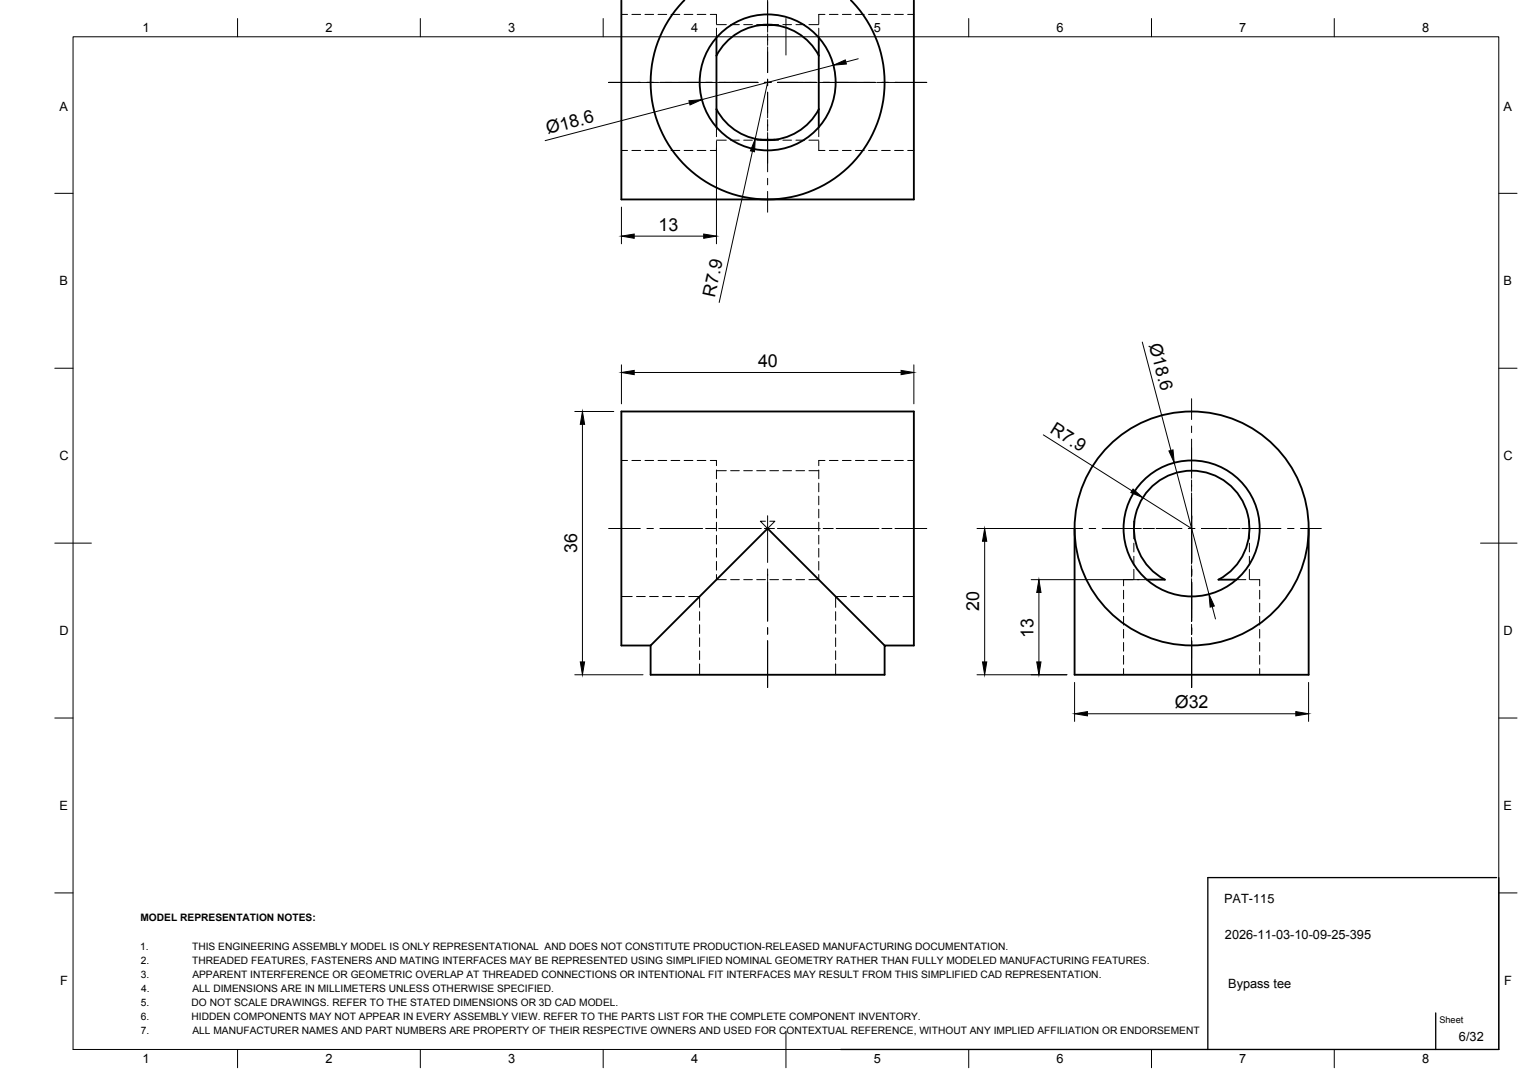
ISO-10303-21;
HEADER;
/* Generated by software containing ST-Developer
 * from STEP Tools, Inc. (www.steptools.com) 
 */

FILE_DESCRIPTION(
/* description */ ('Union bypass pipe loop'),
/* implementation_level */ '2;1');

FILE_NAME(
/* name */ 'Bypass tee.step',
/* time_stamp */ '2026-10-27T21:00:29-07:00',
/* author */ (''),
/* organization */ (''),
/* preprocessor_version */ 'ST-DEVELOPER v20.2',
/* originating_system */ 'Autodesk Translation Framework v15.17.0.0',
/* authorisation */ '');

FILE_SCHEMA (('AUTOMOTIVE_DESIGN { 1 0 10303 214 3 1 1 }'));
ENDSEC;

DATA;
#10=MECHANICAL_DESIGN_GEOMETRIC_PRESENTATION_REPRESENTATION('',(#460),#10095);
#11=ELLIPSE('',#6238,1.31521861300698,0.93);
#12=ELLIPSE('',#6239,1.31521861300698,0.93);
#13=ELLIPSE('',#6241,1.31521861300698,0.93);
#14=ELLIPSE('',#6249,1.11722871427474,0.789999999999999);
#15=ELLIPSE('',#6250,1.11722871427474,0.789999999999999);
#16=ELLIPSE('',#6254,1.11722871427474,0.789999999999999);
#17=ELLIPSE('',#6255,1.11722871427474,0.789999999999999);
#18=ELLIPSE('',#6263,1.11722871427474,0.789999999999999);
#19=ELLIPSE('',#6264,1.11722871427474,0.789999999999999);
#20=ELLIPSE('',#6265,1.11722871427474,0.789999999999999);
#21=ELLIPSE('',#6266,1.11722871427474,0.789999999999999);
#22=ELLIPSE('',#6274,2.26274169979695,1.6);
#23=ELLIPSE('',#6275,2.26274169979695,1.6);
#24=ELLIPSE('',#6277,2.26274169979695,1.6);
#396=SHAPE_REPRESENTATION_RELATIONSHIP('SRR','None',#10265,#428);
#428=ADVANCED_BREP_SHAPE_REPRESENTATION('',(#490),#10077);
#460=STYLED_ITEM('',(#10493),#490);
#490=MANIFOLD_SOLID_BREP('Body1',#5533);
#579=FACE_BOUND('',#1404,.T.);
#580=FACE_BOUND('',#1407,.T.);
#581=FACE_BOUND('',#1409,.T.);
#723=PLANE('',#6233);
#724=PLANE('',#6242);
#725=PLANE('',#6251);
#726=PLANE('',#6256);
#727=PLANE('',#6267);
#728=PLANE('',#6272);
#729=PLANE('',#6278);
#730=PLANE('',#6282);
#731=PLANE('',#6283);
#988=FACE_OUTER_BOUND('',#1388,.T.);
#989=FACE_OUTER_BOUND('',#1389,.T.);
#990=FACE_OUTER_BOUND('',#1390,.T.);
#991=FACE_OUTER_BOUND('',#1391,.T.);
#992=FACE_OUTER_BOUND('',#1392,.T.);
#993=FACE_OUTER_BOUND('',#1393,.T.);
#994=FACE_OUTER_BOUND('',#1394,.T.);
#995=FACE_OUTER_BOUND('',#1395,.T.);
#996=FACE_OUTER_BOUND('',#1396,.T.);
#997=FACE_OUTER_BOUND('',#1397,.T.);
#998=FACE_OUTER_BOUND('',#1398,.T.);
#999=FACE_OUTER_BOUND('',#1399,.T.);
#1000=FACE_OUTER_BOUND('',#1400,.T.);
#1001=FACE_OUTER_BOUND('',#1401,.T.);
#1002=FACE_OUTER_BOUND('',#1402,.T.);
#1003=FACE_OUTER_BOUND('',#1403,.T.);
#1004=FACE_OUTER_BOUND('',#1405,.T.);
#1005=FACE_OUTER_BOUND('',#1406,.T.);
#1006=FACE_OUTER_BOUND('',#1408,.T.);
#1388=EDGE_LOOP('',(#4352,#4353,#4354,#4355));
#1389=EDGE_LOOP('',(#4356,#4357,#4358,#4359,#4360,#4361,#4362,#4363));
#1390=EDGE_LOOP('',(#4364,#4365,#4366,#4367));
#1391=EDGE_LOOP('',(#4368,#4369,#4370,#4371,#4372,#4373));
#1392=EDGE_LOOP('',(#4374,#4375,#4376));
#1393=EDGE_LOOP('',(#4377,#4378,#4379,#4380,#4381));
#1394=EDGE_LOOP('',(#4382,#4383,#4384));
#1395=EDGE_LOOP('',(#4385,#4386,#4387,#4388,#4389));
#1396=EDGE_LOOP('',(#4390,#4391,#4392,#4393,#4394,#4395,#4396));
#1397=EDGE_LOOP('',(#4397,#4398,#4399,#4400,#4401,#4402,#4403,#4404,#4405,
#4406,#4407,#4408));
#1398=EDGE_LOOP('',(#4409,#4410));
#1399=EDGE_LOOP('',(#4411,#4412,#4413));
#1400=EDGE_LOOP('',(#4414,#4415,#4416));
#1401=EDGE_LOOP('',(#4417,#4418));
#1402=EDGE_LOOP('',(#4419,#4420,#4421,#4422,#4423,#4424));
#1403=EDGE_LOOP('',(#4425));
#1404=EDGE_LOOP('',(#4426));
#1405=EDGE_LOOP('',(#4427,#4428,#4429,#4430,#4431,#4432,#4433,#4434,#4435));
#1406=EDGE_LOOP('',(#4436));
#1407=EDGE_LOOP('',(#4437));
#1408=EDGE_LOOP('',(#4438));
#1409=EDGE_LOOP('',(#4439));
#1797=LINE('',#9166,#2173);
#1798=LINE('',#9170,#2174);
#1799=LINE('',#9176,#2175);
#1800=LINE('',#9185,#2176);
#1801=LINE('',#9188,#2177);
#1802=LINE('',#9193,#2178);
#1803=LINE('',#9214,#2179);
#1804=LINE('',#9219,#2180);
#1805=LINE('',#9224,#2181);
#1806=LINE('',#9239,#2182);
#1807=LINE('',#9246,#2183);
#1808=LINE('',#9248,#2184);
#2173=VECTOR('',#7451,1.);
#2174=VECTOR('',#7454,1.);
#2175=VECTOR('',#7461,0.93);
#2176=VECTOR('',#7472,1.);
#2177=VECTOR('',#7475,1.);
#2178=VECTOR('',#7480,0.93);
#2179=VECTOR('',#7513,0.93);
#2180=VECTOR('',#7518,1.);
#2181=VECTOR('',#7523,1.);
#2182=VECTOR('',#7544,1.6);
#2183=VECTOR('',#7555,1.6);
#2184=VECTOR('',#7556,1.6);
#2496=CIRCLE('',#6234,0.93);
#2497=CIRCLE('',#6235,0.789999999999999);
#2498=CIRCLE('',#6237,0.93);
#2499=CIRCLE('',#6240,0.93);
#2500=CIRCLE('',#6243,0.789999999999999);
#2501=CIRCLE('',#6245,0.93);
#2502=CIRCLE('',#6246,0.93);
#2503=CIRCLE('',#6247,0.93);
#2504=CIRCLE('',#6252,0.79);
#2505=CIRCLE('',#6257,0.79);
#2506=CIRCLE('',#6258,0.93);
#2507=CIRCLE('',#6259,0.93);
#2508=CIRCLE('',#6261,0.93);
#2509=CIRCLE('',#6268,0.789999999999999);
#2510=CIRCLE('',#6270,0.789999999999999);
#2511=CIRCLE('',#6276,1.6);
#2512=CIRCLE('',#6280,1.6);
#2513=CIRCLE('',#6281,1.6);
#2832=VERTEX_POINT('',#9164);
#2833=VERTEX_POINT('',#9165);
#2834=VERTEX_POINT('',#9167);
#2835=VERTEX_POINT('',#9169);
#2836=VERTEX_POINT('',#9173);
#2837=VERTEX_POINT('',#9175);
#2838=VERTEX_POINT('',#9178);
#2839=VERTEX_POINT('',#9180);
#2840=VERTEX_POINT('',#9184);
#2841=VERTEX_POINT('',#9186);
#2842=VERTEX_POINT('',#9190);
#2843=VERTEX_POINT('',#9192);
#2844=VERTEX_POINT('',#9197);
#2845=VERTEX_POINT('',#9203);
#2846=VERTEX_POINT('',#9208);
#2847=VERTEX_POINT('',#9212);
#2848=VERTEX_POINT('',#9216);
#2849=VERTEX_POINT('',#9218);
#2850=VERTEX_POINT('',#9221);
#2851=VERTEX_POINT('',#9223);
#2852=VERTEX_POINT('',#9233);
#2853=VERTEX_POINT('',#9234);
#2854=VERTEX_POINT('',#9236);
#2855=VERTEX_POINT('',#9238);
#2856=VERTEX_POINT('',#9244);
#2857=VERTEX_POINT('',#9247);
#3374=EDGE_CURVE('',#2832,#2833,#1797,.T.);
#3375=EDGE_CURVE('',#2834,#2832,#2496,.T.);
#3376=EDGE_CURVE('',#2835,#2834,#1798,.T.);
#3377=EDGE_CURVE('',#2833,#2835,#2497,.T.);
#3378=EDGE_CURVE('',#2836,#2836,#2498,.T.);
#3379=EDGE_CURVE('',#2836,#2837,#1799,.T.);
#3380=EDGE_CURVE('',#2834,#2837,#11,.T.);
#3381=EDGE_CURVE('',#2838,#2832,#12,.T.);
#3382=EDGE_CURVE('',#2838,#2839,#2499,.T.);
#3383=EDGE_CURVE('',#2837,#2839,#13,.T.);
#3384=EDGE_CURVE('',#2840,#2838,#1800,.T.);
#3385=EDGE_CURVE('',#2841,#2840,#2500,.T.);
#3386=EDGE_CURVE('',#2839,#2841,#1801,.T.);
#3387=EDGE_CURVE('',#2842,#2832,#2501,.T.);
#3388=EDGE_CURVE('',#2842,#2843,#1802,.T.);
#3389=EDGE_CURVE('',#2843,#2843,#2502,.T.);
#3390=EDGE_CURVE('',#2838,#2842,#2503,.T.);
#3391=EDGE_CURVE('',#2844,#2835,#14,.T.);
#3392=EDGE_CURVE('',#2833,#2844,#15,.T.);
#3393=EDGE_CURVE('',#2840,#2833,#2504,.T.);
#3394=EDGE_CURVE('',#2845,#2840,#16,.T.);
#3395=EDGE_CURVE('',#2841,#2845,#17,.T.);
#3396=EDGE_CURVE('',#2835,#2841,#2505,.T.);
#3397=EDGE_CURVE('',#2846,#2834,#2506,.T.);
#3398=EDGE_CURVE('',#2839,#2846,#2507,.T.);
#3399=EDGE_CURVE('',#2847,#2847,#2508,.T.);
#3400=EDGE_CURVE('',#2847,#2846,#1803,.T.);
#3401=EDGE_CURVE('',#2844,#2848,#18,.T.);
#3402=EDGE_CURVE('',#2848,#2849,#1804,.T.);
#3403=EDGE_CURVE('',#2849,#2844,#19,.T.);
#3404=EDGE_CURVE('',#2845,#2850,#20,.T.);
#3405=EDGE_CURVE('',#2850,#2851,#1805,.T.);
#3406=EDGE_CURVE('',#2851,#2845,#21,.T.);
#3407=EDGE_CURVE('',#2851,#2850,#2509,.T.);
#3408=EDGE_CURVE('',#2849,#2848,#2510,.T.);
#3409=EDGE_CURVE('',#2852,#2853,#22,.T.);
#3410=EDGE_CURVE('',#2854,#2852,#23,.T.);
#3411=EDGE_CURVE('',#2854,#2855,#1806,.T.);
#3412=EDGE_CURVE('',#2855,#2855,#2511,.T.);
#3413=EDGE_CURVE('',#2853,#2854,#24,.T.);
#3414=EDGE_CURVE('',#2856,#2856,#2512,.T.);
#3415=EDGE_CURVE('',#2856,#2852,#1807,.T.);
#3416=EDGE_CURVE('',#2852,#2857,#1808,.T.);
#3417=EDGE_CURVE('',#2857,#2857,#2513,.T.);
#4352=ORIENTED_EDGE('',*,*,#3374,.F.);
#4353=ORIENTED_EDGE('',*,*,#3375,.F.);
#4354=ORIENTED_EDGE('',*,*,#3376,.F.);
#4355=ORIENTED_EDGE('',*,*,#3377,.F.);
#4356=ORIENTED_EDGE('',*,*,#3378,.F.);
#4357=ORIENTED_EDGE('',*,*,#3379,.T.);
#4358=ORIENTED_EDGE('',*,*,#3380,.F.);
#4359=ORIENTED_EDGE('',*,*,#3375,.T.);
#4360=ORIENTED_EDGE('',*,*,#3381,.F.);
#4361=ORIENTED_EDGE('',*,*,#3382,.T.);
#4362=ORIENTED_EDGE('',*,*,#3383,.F.);
#4363=ORIENTED_EDGE('',*,*,#3379,.F.);
#4364=ORIENTED_EDGE('',*,*,#3384,.F.);
#4365=ORIENTED_EDGE('',*,*,#3385,.F.);
#4366=ORIENTED_EDGE('',*,*,#3386,.F.);
#4367=ORIENTED_EDGE('',*,*,#3382,.F.);
#4368=ORIENTED_EDGE('',*,*,#3381,.T.);
#4369=ORIENTED_EDGE('',*,*,#3387,.F.);
#4370=ORIENTED_EDGE('',*,*,#3388,.T.);
#4371=ORIENTED_EDGE('',*,*,#3389,.F.);
#4372=ORIENTED_EDGE('',*,*,#3388,.F.);
#4373=ORIENTED_EDGE('',*,*,#3390,.F.);
#4374=ORIENTED_EDGE('',*,*,#3377,.T.);
#4375=ORIENTED_EDGE('',*,*,#3391,.F.);
#4376=ORIENTED_EDGE('',*,*,#3392,.F.);
#4377=ORIENTED_EDGE('',*,*,#3384,.T.);
#4378=ORIENTED_EDGE('',*,*,#3390,.T.);
#4379=ORIENTED_EDGE('',*,*,#3387,.T.);
#4380=ORIENTED_EDGE('',*,*,#3374,.T.);
#4381=ORIENTED_EDGE('',*,*,#3393,.F.);
#4382=ORIENTED_EDGE('',*,*,#3385,.T.);
#4383=ORIENTED_EDGE('',*,*,#3394,.F.);
#4384=ORIENTED_EDGE('',*,*,#3395,.F.);
#4385=ORIENTED_EDGE('',*,*,#3386,.T.);
#4386=ORIENTED_EDGE('',*,*,#3396,.F.);
#4387=ORIENTED_EDGE('',*,*,#3376,.T.);
#4388=ORIENTED_EDGE('',*,*,#3397,.F.);
#4389=ORIENTED_EDGE('',*,*,#3398,.F.);
#4390=ORIENTED_EDGE('',*,*,#3399,.F.);
#4391=ORIENTED_EDGE('',*,*,#3400,.T.);
#4392=ORIENTED_EDGE('',*,*,#3397,.T.);
#4393=ORIENTED_EDGE('',*,*,#3380,.T.);
#4394=ORIENTED_EDGE('',*,*,#3383,.T.);
#4395=ORIENTED_EDGE('',*,*,#3398,.T.);
#4396=ORIENTED_EDGE('',*,*,#3400,.F.);
#4397=ORIENTED_EDGE('',*,*,#3393,.T.);
#4398=ORIENTED_EDGE('',*,*,#3392,.T.);
#4399=ORIENTED_EDGE('',*,*,#3401,.T.);
#4400=ORIENTED_EDGE('',*,*,#3402,.T.);
#4401=ORIENTED_EDGE('',*,*,#3403,.T.);
#4402=ORIENTED_EDGE('',*,*,#3391,.T.);
#4403=ORIENTED_EDGE('',*,*,#3396,.T.);
#4404=ORIENTED_EDGE('',*,*,#3395,.T.);
#4405=ORIENTED_EDGE('',*,*,#3404,.T.);
#4406=ORIENTED_EDGE('',*,*,#3405,.T.);
#4407=ORIENTED_EDGE('',*,*,#3406,.T.);
#4408=ORIENTED_EDGE('',*,*,#3394,.T.);
#4409=ORIENTED_EDGE('',*,*,#3405,.F.);
#4410=ORIENTED_EDGE('',*,*,#3407,.F.);
#4411=ORIENTED_EDGE('',*,*,#3403,.F.);
#4412=ORIENTED_EDGE('',*,*,#3408,.T.);
#4413=ORIENTED_EDGE('',*,*,#3401,.F.);
#4414=ORIENTED_EDGE('',*,*,#3406,.F.);
#4415=ORIENTED_EDGE('',*,*,#3407,.T.);
#4416=ORIENTED_EDGE('',*,*,#3404,.F.);
#4417=ORIENTED_EDGE('',*,*,#3402,.F.);
#4418=ORIENTED_EDGE('',*,*,#3408,.F.);
#4419=ORIENTED_EDGE('',*,*,#3409,.F.);
#4420=ORIENTED_EDGE('',*,*,#3410,.F.);
#4421=ORIENTED_EDGE('',*,*,#3411,.T.);
#4422=ORIENTED_EDGE('',*,*,#3412,.T.);
#4423=ORIENTED_EDGE('',*,*,#3411,.F.);
#4424=ORIENTED_EDGE('',*,*,#3413,.F.);
#4425=ORIENTED_EDGE('',*,*,#3412,.F.);
#4426=ORIENTED_EDGE('',*,*,#3378,.T.);
#4427=ORIENTED_EDGE('',*,*,#3414,.F.);
#4428=ORIENTED_EDGE('',*,*,#3415,.T.);
#4429=ORIENTED_EDGE('',*,*,#3409,.T.);
#4430=ORIENTED_EDGE('',*,*,#3413,.T.);
#4431=ORIENTED_EDGE('',*,*,#3410,.T.);
#4432=ORIENTED_EDGE('',*,*,#3416,.T.);
#4433=ORIENTED_EDGE('',*,*,#3417,.T.);
#4434=ORIENTED_EDGE('',*,*,#3416,.F.);
#4435=ORIENTED_EDGE('',*,*,#3415,.F.);
#4436=ORIENTED_EDGE('',*,*,#3414,.T.);
#4437=ORIENTED_EDGE('',*,*,#3389,.T.);
#4438=ORIENTED_EDGE('',*,*,#3417,.F.);
#4439=ORIENTED_EDGE('',*,*,#3399,.T.);
#5131=CYLINDRICAL_SURFACE('',#6236,0.93);
#5132=CYLINDRICAL_SURFACE('',#6244,0.93);
#5133=CYLINDRICAL_SURFACE('',#6248,0.789999999999999);
#5134=CYLINDRICAL_SURFACE('',#6253,0.789999999999999);
#5135=CYLINDRICAL_SURFACE('',#6260,0.93);
#5136=CYLINDRICAL_SURFACE('',#6262,0.79);
#5137=CYLINDRICAL_SURFACE('',#6269,0.789999999999999);
#5138=CYLINDRICAL_SURFACE('',#6271,0.789999999999999);
#5139=CYLINDRICAL_SURFACE('',#6273,1.6);
#5140=CYLINDRICAL_SURFACE('',#6279,1.6);
#5337=ADVANCED_FACE('',(#988),#723,.F.);
#5338=ADVANCED_FACE('',(#989),#5131,.F.);
#5339=ADVANCED_FACE('',(#990),#724,.F.);
#5340=ADVANCED_FACE('',(#991),#5132,.F.);
#5341=ADVANCED_FACE('',(#992),#5133,.F.);
#5342=ADVANCED_FACE('',(#993),#725,.T.);
#5343=ADVANCED_FACE('',(#994),#5134,.F.);
#5344=ADVANCED_FACE('',(#995),#726,.F.);
#5345=ADVANCED_FACE('',(#996),#5135,.F.);
#5346=ADVANCED_FACE('',(#997),#5136,.F.);
#5347=ADVANCED_FACE('',(#998),#727,.F.);
#5348=ADVANCED_FACE('',(#999),#5137,.F.);
#5349=ADVANCED_FACE('',(#1000),#5138,.F.);
#5350=ADVANCED_FACE('',(#1001),#728,.F.);
#5351=ADVANCED_FACE('',(#1002),#5139,.T.);
#5352=ADVANCED_FACE('',(#1003,#579),#729,.F.);
#5353=ADVANCED_FACE('',(#1004),#5140,.T.);
#5354=ADVANCED_FACE('',(#1005,#580),#730,.T.);
#5355=ADVANCED_FACE('',(#1006,#581),#731,.F.);
#5533=CLOSED_SHELL('',(#5337,#5338,#5339,#5340,#5341,#5342,#5343,#5344,
#5345,#5346,#5347,#5348,#5349,#5350,#5351,#5352,#5353,#5354,#5355));
#6232=AXIS2_PLACEMENT_3D('',#9162,#7447,#7448);
#6233=AXIS2_PLACEMENT_3D('',#9163,#7449,#7450);
#6234=AXIS2_PLACEMENT_3D('',#9168,#7452,#7453);
#6235=AXIS2_PLACEMENT_3D('',#9171,#7455,#7456);
#6236=AXIS2_PLACEMENT_3D('',#9172,#7457,#7458);
#6237=AXIS2_PLACEMENT_3D('',#9174,#7459,#7460);
#6238=AXIS2_PLACEMENT_3D('',#9177,#7462,#7463);
#6239=AXIS2_PLACEMENT_3D('',#9179,#7464,#7465);
#6240=AXIS2_PLACEMENT_3D('',#9181,#7466,#7467);
#6241=AXIS2_PLACEMENT_3D('',#9182,#7468,#7469);
#6242=AXIS2_PLACEMENT_3D('',#9183,#7470,#7471);
#6243=AXIS2_PLACEMENT_3D('',#9187,#7473,#7474);
#6244=AXIS2_PLACEMENT_3D('',#9189,#7476,#7477);
#6245=AXIS2_PLACEMENT_3D('',#9191,#7478,#7479);
#6246=AXIS2_PLACEMENT_3D('',#9194,#7481,#7482);
#6247=AXIS2_PLACEMENT_3D('',#9195,#7483,#7484);
#6248=AXIS2_PLACEMENT_3D('',#9196,#7485,#7486);
#6249=AXIS2_PLACEMENT_3D('',#9198,#7487,#7488);
#6250=AXIS2_PLACEMENT_3D('',#9199,#7489,#7490);
#6251=AXIS2_PLACEMENT_3D('',#9200,#7491,#7492);
#6252=AXIS2_PLACEMENT_3D('',#9201,#7493,#7494);
#6253=AXIS2_PLACEMENT_3D('',#9202,#7495,#7496);
#6254=AXIS2_PLACEMENT_3D('',#9204,#7497,#7498);
#6255=AXIS2_PLACEMENT_3D('',#9205,#7499,#7500);
#6256=AXIS2_PLACEMENT_3D('',#9206,#7501,#7502);
#6257=AXIS2_PLACEMENT_3D('',#9207,#7503,#7504);
#6258=AXIS2_PLACEMENT_3D('',#9209,#7505,#7506);
#6259=AXIS2_PLACEMENT_3D('',#9210,#7507,#7508);
#6260=AXIS2_PLACEMENT_3D('',#9211,#7509,#7510);
#6261=AXIS2_PLACEMENT_3D('',#9213,#7511,#7512);
#6262=AXIS2_PLACEMENT_3D('',#9215,#7514,#7515);
#6263=AXIS2_PLACEMENT_3D('',#9217,#7516,#7517);
#6264=AXIS2_PLACEMENT_3D('',#9220,#7519,#7520);
#6265=AXIS2_PLACEMENT_3D('',#9222,#7521,#7522);
#6266=AXIS2_PLACEMENT_3D('',#9225,#7524,#7525);
#6267=AXIS2_PLACEMENT_3D('',#9226,#7526,#7527);
#6268=AXIS2_PLACEMENT_3D('',#9227,#7528,#7529);
#6269=AXIS2_PLACEMENT_3D('',#9228,#7530,#7531);
#6270=AXIS2_PLACEMENT_3D('',#9229,#7532,#7533);
#6271=AXIS2_PLACEMENT_3D('',#9230,#7534,#7535);
#6272=AXIS2_PLACEMENT_3D('',#9231,#7536,#7537);
#6273=AXIS2_PLACEMENT_3D('',#9232,#7538,#7539);
#6274=AXIS2_PLACEMENT_3D('',#9235,#7540,#7541);
#6275=AXIS2_PLACEMENT_3D('',#9237,#7542,#7543);
#6276=AXIS2_PLACEMENT_3D('',#9240,#7545,#7546);
#6277=AXIS2_PLACEMENT_3D('',#9241,#7547,#7548);
#6278=AXIS2_PLACEMENT_3D('',#9242,#7549,#7550);
#6279=AXIS2_PLACEMENT_3D('',#9243,#7551,#7552);
#6280=AXIS2_PLACEMENT_3D('',#9245,#7553,#7554);
#6281=AXIS2_PLACEMENT_3D('',#9249,#7557,#7558);
#6282=AXIS2_PLACEMENT_3D('',#9250,#7559,#7560);
#6283=AXIS2_PLACEMENT_3D('',#9251,#7561,#7562);
#7447=DIRECTION('axis',(0.,0.,1.));
#7448=DIRECTION('refdir',(1.,0.,0.));
#7449=DIRECTION('center_axis',(0.,1.,0.));
#7450=DIRECTION('ref_axis',(1.,0.,0.));
#7451=DIRECTION('',(0.,0.,-1.));
#7452=DIRECTION('center_axis',(0.,1.,0.));
#7453=DIRECTION('ref_axis',(1.,0.,0.));
#7454=DIRECTION('',(0.,0.,1.));
#7455=DIRECTION('center_axis',(0.,-1.,0.));
#7456=DIRECTION('ref_axis',(1.,0.,0.));
#7457=DIRECTION('center_axis',(0.,1.,0.));
#7458=DIRECTION('ref_axis',(1.,0.,0.));
#7459=DIRECTION('center_axis',(0.,1.,0.));
#7460=DIRECTION('ref_axis',(1.,0.,0.));
#7461=DIRECTION('',(0.,1.,0.));
#7462=DIRECTION('center_axis',(0.707106781186548,-0.707106781186548,0.));
#7463=DIRECTION('ref_axis',(0.707106781186547,0.707106781186547,0.));
#7464=DIRECTION('center_axis',(-0.707106781186548,-0.707106781186548,0.));
#7465=DIRECTION('ref_axis',(0.707106781186547,-0.707106781186547,0.));
#7466=DIRECTION('center_axis',(0.,1.,0.));
#7467=DIRECTION('ref_axis',(1.,0.,0.));
#7468=DIRECTION('center_axis',(0.707106781186548,-0.707106781186548,0.));
#7469=DIRECTION('ref_axis',(0.707106781186547,0.707106781186547,0.));
#7470=DIRECTION('center_axis',(0.,1.,0.));
#7471=DIRECTION('ref_axis',(1.,0.,0.));
#7472=DIRECTION('',(0.,0.,-1.));
#7473=DIRECTION('center_axis',(0.,-1.,0.));
#7474=DIRECTION('ref_axis',(1.,0.,0.));
#7475=DIRECTION('',(0.,0.,1.));
#7476=DIRECTION('center_axis',(1.,0.,0.));
#7477=DIRECTION('ref_axis',(0.,0.,-1.));
#7478=DIRECTION('center_axis',(1.,0.,0.));
#7479=DIRECTION('ref_axis',(0.,0.,-1.));
#7480=DIRECTION('',(1.,0.,0.));
#7481=DIRECTION('center_axis',(-1.,0.,0.));
#7482=DIRECTION('ref_axis',(0.,0.,-1.));
#7483=DIRECTION('center_axis',(1.,0.,0.));
#7484=DIRECTION('ref_axis',(0.,0.,-1.));
#7485=DIRECTION('center_axis',(0.,1.,0.));
#7486=DIRECTION('ref_axis',(1.,0.,0.));
#7487=DIRECTION('center_axis',(0.707106781186548,-0.707106781186547,0.));
#7488=DIRECTION('ref_axis',(0.707106781186547,0.707106781186548,0.));
#7489=DIRECTION('center_axis',(-0.707106781186548,-0.707106781186547,0.));
#7490=DIRECTION('ref_axis',(0.707106781186547,-0.707106781186548,0.));
#7491=DIRECTION('center_axis',(1.,0.,0.));
#7492=DIRECTION('ref_axis',(0.,0.,-1.));
#7493=DIRECTION('center_axis',(1.,0.,0.));
#7494=DIRECTION('ref_axis',(0.,0.,-1.));
#7495=DIRECTION('center_axis',(0.,1.,0.));
#7496=DIRECTION('ref_axis',(1.,0.,0.));
#7497=DIRECTION('center_axis',(-0.707106781186548,-0.707106781186547,0.));
#7498=DIRECTION('ref_axis',(0.707106781186547,-0.707106781186548,0.));
#7499=DIRECTION('center_axis',(0.707106781186548,-0.707106781186547,0.));
#7500=DIRECTION('ref_axis',(0.707106781186547,0.707106781186548,0.));
#7501=DIRECTION('center_axis',(1.,0.,0.));
#7502=DIRECTION('ref_axis',(0.,0.,-1.));
#7503=DIRECTION('center_axis',(-1.,0.,0.));
#7504=DIRECTION('ref_axis',(0.,0.,-1.));
#7505=DIRECTION('center_axis',(1.,0.,0.));
#7506=DIRECTION('ref_axis',(0.,0.,-1.));
#7507=DIRECTION('center_axis',(1.,0.,0.));
#7508=DIRECTION('ref_axis',(0.,0.,-1.));
#7509=DIRECTION('center_axis',(1.,0.,0.));
#7510=DIRECTION('ref_axis',(0.,0.,-1.));
#7511=DIRECTION('center_axis',(1.,0.,0.));
#7512=DIRECTION('ref_axis',(0.,0.,-1.));
#7513=DIRECTION('',(1.,0.,0.));
#7514=DIRECTION('center_axis',(1.,0.,0.));
#7515=DIRECTION('ref_axis',(0.,1.,1.60812264967664E-16));
#7516=DIRECTION('center_axis',(-0.707106781186548,0.707106781186547,0.));
#7517=DIRECTION('ref_axis',(0.707106781186547,0.707106781186548,0.));
#7518=DIRECTION('',(-1.,0.,0.));
#7519=DIRECTION('center_axis',(0.707106781186548,0.707106781186547,0.));
#7520=DIRECTION('ref_axis',(0.707106781186547,-0.707106781186548,0.));
#7521=DIRECTION('center_axis',(0.707106781186548,0.707106781186547,0.));
#7522=DIRECTION('ref_axis',(0.707106781186547,-0.707106781186548,0.));
#7523=DIRECTION('',(1.,0.,0.));
#7524=DIRECTION('center_axis',(-0.707106781186548,0.707106781186547,0.));
#7525=DIRECTION('ref_axis',(0.707106781186547,0.707106781186548,0.));
#7526=DIRECTION('center_axis',(0.,1.,0.));
#7527=DIRECTION('ref_axis',(1.,0.,0.));
#7528=DIRECTION('center_axis',(0.,1.,0.));
#7529=DIRECTION('ref_axis',(1.,0.,0.));
#7530=DIRECTION('center_axis',(0.,1.,0.));
#7531=DIRECTION('ref_axis',(1.,0.,0.));
#7532=DIRECTION('center_axis',(0.,1.,0.));
#7533=DIRECTION('ref_axis',(1.,0.,0.));
#7534=DIRECTION('center_axis',(0.,1.,0.));
#7535=DIRECTION('ref_axis',(1.,0.,0.));
#7536=DIRECTION('center_axis',(0.,1.,0.));
#7537=DIRECTION('ref_axis',(1.,0.,0.));
#7538=DIRECTION('center_axis',(0.,1.,0.));
#7539=DIRECTION('ref_axis',(1.,0.,0.));
#7540=DIRECTION('center_axis',(0.707106781186548,0.707106781186547,0.));
#7541=DIRECTION('ref_axis',(0.707106781186547,-0.707106781186548,0.));
#7542=DIRECTION('center_axis',(-0.707106781186548,0.707106781186547,0.));
#7543=DIRECTION('ref_axis',(0.707106781186547,0.707106781186548,0.));
#7544=DIRECTION('',(0.,-1.,0.));
#7545=DIRECTION('center_axis',(0.,1.,0.));
#7546=DIRECTION('ref_axis',(1.,0.,0.));
#7547=DIRECTION('center_axis',(-0.707106781186548,0.707106781186547,0.));
#7548=DIRECTION('ref_axis',(0.707106781186547,0.707106781186548,0.));
#7549=DIRECTION('center_axis',(0.,1.,0.));
#7550=DIRECTION('ref_axis',(1.,0.,0.));
#7551=DIRECTION('center_axis',(1.,0.,0.));
#7552=DIRECTION('ref_axis',(0.,0.,-1.));
#7553=DIRECTION('center_axis',(1.,0.,0.));
#7554=DIRECTION('ref_axis',(0.,0.,-1.));
#7555=DIRECTION('',(-1.,0.,0.));
#7556=DIRECTION('',(-1.,0.,0.));
#7557=DIRECTION('center_axis',(1.,0.,0.));
#7558=DIRECTION('ref_axis',(0.,0.,-1.));
#7559=DIRECTION('center_axis',(1.,0.,0.));
#7560=DIRECTION('ref_axis',(0.,0.,-1.));
#7561=DIRECTION('center_axis',(1.,0.,0.));
#7562=DIRECTION('ref_axis',(0.,0.,-1.));
#9162=CARTESIAN_POINT('',(0.,0.,0.));
#9163=CARTESIAN_POINT('Origin',(-12.,-0.7,5.));
#9164=CARTESIAN_POINT('',(-11.3,-0.7,5.61229078059367));
#9165=CARTESIAN_POINT('',(-11.3,-0.700000000000001,5.36619666847201));
#9166=CARTESIAN_POINT('',(-11.3,-0.7,5.));
#9167=CARTESIAN_POINT('',(-12.7,-0.7,5.61229078059366));
#9168=CARTESIAN_POINT('Origin',(-12.,-0.7,5.));
#9169=CARTESIAN_POINT('',(-12.7,-0.700000000000002,5.36619666847201));
#9170=CARTESIAN_POINT('',(-12.7,-0.7,5.));
#9171=CARTESIAN_POINT('Origin',(-12.,-0.7,5.));
#9172=CARTESIAN_POINT('Origin',(-12.,-2.1,5.));
#9173=CARTESIAN_POINT('',(-12.93,-2.,5.));
#9174=CARTESIAN_POINT('Origin',(-12.,-2.,5.));
#9175=CARTESIAN_POINT('',(-12.93,-0.93,5.));
#9176=CARTESIAN_POINT('',(-12.93,-2.1,5.));
#9177=CARTESIAN_POINT('Origin',(-12.,0.,5.));
#9178=CARTESIAN_POINT('',(-11.3,-0.7,4.38770921940633));
#9179=CARTESIAN_POINT('Origin',(-12.,0.,5.));
#9180=CARTESIAN_POINT('',(-12.7,-0.7,4.38770921940634));
#9181=CARTESIAN_POINT('Origin',(-12.,-0.7,5.));
#9182=CARTESIAN_POINT('Origin',(-12.,0.,5.));
#9183=CARTESIAN_POINT('Origin',(-12.,-0.7,5.));
#9184=CARTESIAN_POINT('',(-11.3,-0.700000000000001,4.63380333152799));
#9185=CARTESIAN_POINT('',(-11.3,-0.7,5.));
#9186=CARTESIAN_POINT('',(-12.7,-0.700000000000002,4.63380333152799));
#9187=CARTESIAN_POINT('Origin',(-12.,-0.7,5.));
#9188=CARTESIAN_POINT('',(-12.7,-0.7,5.));
#9189=CARTESIAN_POINT('Origin',(-11.3,0.,5.));
#9190=CARTESIAN_POINT('',(-11.3,-1.13892152320704E-16,5.93));
#9191=CARTESIAN_POINT('Origin',(-11.3,0.,5.));
#9192=CARTESIAN_POINT('',(-10.,1.13892152320704E-16,5.93));
#9193=CARTESIAN_POINT('',(-11.3,-1.13892152320704E-16,5.93));
#9194=CARTESIAN_POINT('Origin',(-10.,0.,5.));
#9195=CARTESIAN_POINT('Origin',(-11.3,0.,5.));
#9196=CARTESIAN_POINT('Origin',(-12.,-2.1,5.));
#9197=CARTESIAN_POINT('',(-12.,0.,5.79));
#9198=CARTESIAN_POINT('Origin',(-12.,0.,5.));
#9199=CARTESIAN_POINT('Origin',(-12.,0.,5.));
#9200=CARTESIAN_POINT('Origin',(-11.3,0.,5.));
#9201=CARTESIAN_POINT('Origin',(-11.3,0.,5.));
#9202=CARTESIAN_POINT('Origin',(-12.,-2.1,5.));
#9203=CARTESIAN_POINT('',(-12.,0.,4.21));
#9204=CARTESIAN_POINT('Origin',(-12.,0.,5.));
#9205=CARTESIAN_POINT('Origin',(-12.,0.,5.));
#9206=CARTESIAN_POINT('Origin',(-12.7,0.,5.));
#9207=CARTESIAN_POINT('Origin',(-12.7,0.,5.));
#9208=CARTESIAN_POINT('',(-12.7,-1.13892152320704E-16,5.93));
#9209=CARTESIAN_POINT('Origin',(-12.7,0.,5.));
#9210=CARTESIAN_POINT('Origin',(-12.7,0.,5.));
#9211=CARTESIAN_POINT('Origin',(-14.1,0.,5.));
#9212=CARTESIAN_POINT('',(-14.,-1.13892152320704E-16,5.93));
#9213=CARTESIAN_POINT('Origin',(-14.,0.,5.));
#9214=CARTESIAN_POINT('',(-14.1,-1.13892152320704E-16,5.93));
#9215=CARTESIAN_POINT('Origin',(-14.1,0.,5.));
#9216=CARTESIAN_POINT('',(-11.9,0.1,5.7836453279386));
#9217=CARTESIAN_POINT('Origin',(-12.,0.,5.));
#9218=CARTESIAN_POINT('',(-12.1,0.1,5.7836453279386));
#9219=CARTESIAN_POINT('',(-14.1,0.1,5.7836453279386));
#9220=CARTESIAN_POINT('Origin',(-12.,0.,5.));
#9221=CARTESIAN_POINT('',(-12.1,0.1,4.2163546720614));
#9222=CARTESIAN_POINT('Origin',(-12.,0.,5.));
#9223=CARTESIAN_POINT('',(-11.9,0.1,4.2163546720614));
#9224=CARTESIAN_POINT('',(-14.1,0.1,4.2163546720614));
#9225=CARTESIAN_POINT('Origin',(-12.,0.,5.));
#9226=CARTESIAN_POINT('Origin',(-12.,0.1,5.));
#9227=CARTESIAN_POINT('Origin',(-12.,0.1,5.));
#9228=CARTESIAN_POINT('Origin',(-12.,-2.1,5.));
#9229=CARTESIAN_POINT('Origin',(-12.,0.1,5.));
#9230=CARTESIAN_POINT('Origin',(-12.,-2.1,5.));
#9231=CARTESIAN_POINT('Origin',(-12.,0.1,5.));
#9232=CARTESIAN_POINT('Origin',(-12.,-2.,5.));
#9233=CARTESIAN_POINT('',(-12.,0.,6.6));
#9234=CARTESIAN_POINT('',(-12.,0.,3.4));
#9235=CARTESIAN_POINT('Origin',(-12.,0.,5.));
#9236=CARTESIAN_POINT('',(-13.6,-1.6,5.));
#9237=CARTESIAN_POINT('Origin',(-12.,0.,5.));
#9238=CARTESIAN_POINT('',(-13.6,-2.,5.));
#9239=CARTESIAN_POINT('',(-13.6,-2.,5.));
#9240=CARTESIAN_POINT('Origin',(-12.,-2.,5.));
#9241=CARTESIAN_POINT('Origin',(-12.,0.,5.));
#9242=CARTESIAN_POINT('Origin',(-12.,-2.,5.));
#9243=CARTESIAN_POINT('Origin',(-14.,0.,5.));
#9244=CARTESIAN_POINT('',(-10.,-1.95943487863577E-16,6.6));
#9245=CARTESIAN_POINT('Origin',(-10.,0.,5.));
#9246=CARTESIAN_POINT('',(-14.,-1.95943487863577E-16,6.6));
#9247=CARTESIAN_POINT('',(-14.,-1.95943487863577E-16,6.6));
#9248=CARTESIAN_POINT('',(-14.,-1.95943487863577E-16,6.6));
#9249=CARTESIAN_POINT('Origin',(-14.,0.,5.));
#9250=CARTESIAN_POINT('Origin',(-10.,0.,5.));
#9251=CARTESIAN_POINT('Origin',(-14.,0.,5.));
#10040=UNCERTAINTY_MEASURE_WITH_UNIT(LENGTH_MEASURE(0.001),#10096,
'DISTANCE_ACCURACY_VALUE',
'Maximum model space distance between geometric entities at asserted c
onnectivities');
#10058=UNCERTAINTY_MEASURE_WITH_UNIT(LENGTH_MEASURE(0.001),#10096,
'DISTANCE_ACCURACY_VALUE',
'Maximum model space distance between geometric entities at asserted c
onnectivities');
#10077=(
GEOMETRIC_REPRESENTATION_CONTEXT(3)
GLOBAL_UNCERTAINTY_ASSIGNED_CONTEXT((#10040))
GLOBAL_UNIT_ASSIGNED_CONTEXT((#10096,#10098,#10099))
REPRESENTATION_CONTEXT('','3D')
);
#10095=(
GEOMETRIC_REPRESENTATION_CONTEXT(3)
GLOBAL_UNCERTAINTY_ASSIGNED_CONTEXT((#10058))
GLOBAL_UNIT_ASSIGNED_CONTEXT((#10096,#10098,#10099))
REPRESENTATION_CONTEXT('','3D')
);
#10096=(
LENGTH_UNIT()
NAMED_UNIT(*)
SI_UNIT(.CENTI.,.METRE.)
);
#10098=(
NAMED_UNIT(*)
PLANE_ANGLE_UNIT()
SI_UNIT($,.RADIAN.)
);
#10099=(
NAMED_UNIT(*)
SI_UNIT($,.STERADIAN.)
SOLID_ANGLE_UNIT()
);
#10118=SHAPE_DEFINITION_REPRESENTATION(#10189,#10265);
#10189=PRODUCT_DEFINITION_SHAPE('',$,#10302);
#10265=SHAPE_REPRESENTATION('',(#6232),#10077);
#10283=PRODUCT_DEFINITION_CONTEXT('part definition',#10393,'design');
#10302=PRODUCT_DEFINITION('Bypass tee','Bypass tee',#10338,#10283);
#10338=PRODUCT_DEFINITION_FORMATION('',$,#10413);
#10393=APPLICATION_CONTEXT(
'Core Data for Automotive Mechanical Design Process');
#10394=PRODUCT_CONTEXT('part definition',#10393,'mechanical');
#10413=PRODUCT('Bypass tee','Bypass tee','Bypass tee',(#10394));
#10487=COLOUR_RGB('Sky Blue',0.24,0.69,0.87);
#10488=FILL_AREA_STYLE_COLOUR('',#10487);
#10489=FILL_AREA_STYLE('',(#10488));
#10490=SURFACE_STYLE_FILL_AREA(#10489);
#10491=SURFACE_SIDE_STYLE('',(#10490));
#10492=SURFACE_STYLE_USAGE(.BOTH.,#10491);
#10493=PRESENTATION_STYLE_ASSIGNMENT((#10492));
ENDSEC;
END-ISO-10303-21;
